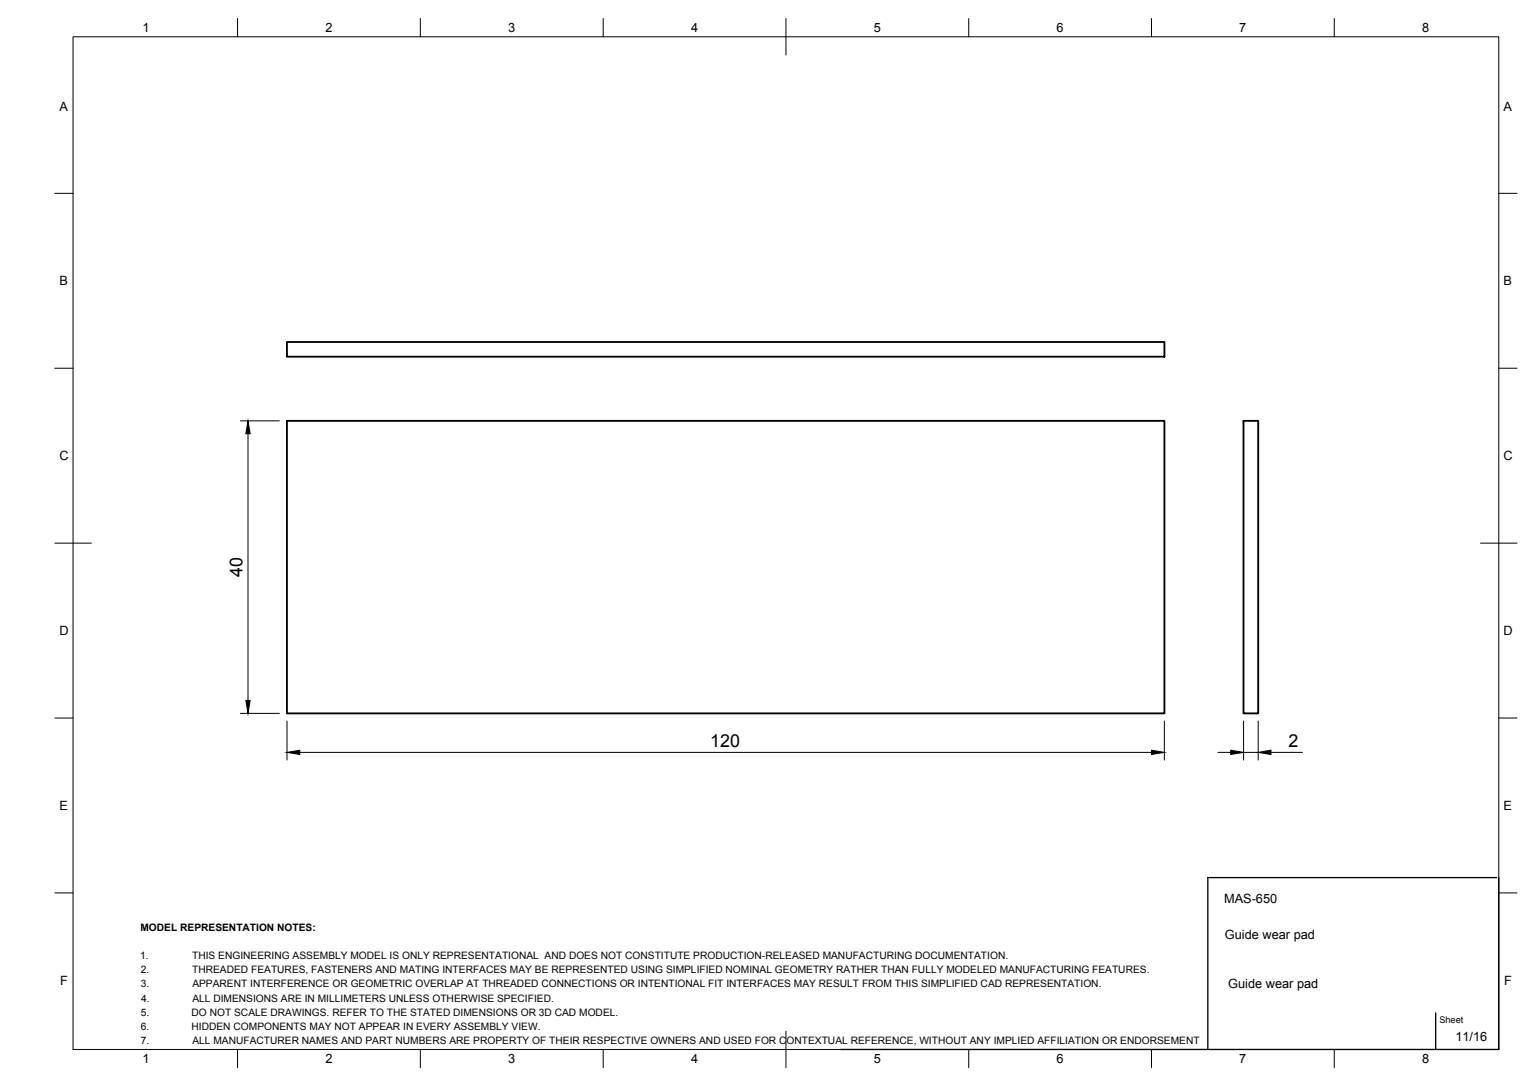
ISO-10303-21;
HEADER;
/* Generated by software containing ST-Developer
 * from STEP Tools, Inc. (www.steptools.com) 
 */

FILE_DESCRIPTION(
/* description */ ('Independent manual traversing gantry with native reusable aluminum pr
ofiles,180mm captured carriage travel, four bronze-bushed rollers, lin
ked ideal rolling motion, bonded acetal lateral guides, positive welde
d end stops and fully retained axle stacks. Editable native profile cu
t lengths220/400mm. Tool attachments viaM6 bridge-plate taps; mounted 
tool outside assembly. Welds, anchors, adhesives, fits, traction, load
/speed/structural/life ratings unassigned.'),
/* implementation_level */ '2;1');

FILE_NAME(
/* name */ 'Guide wear pad.step',
/* time_stamp */ '2026-11-09T20:04:38-08:00',
/* author */ (''),
/* organization */ (''),
/* preprocessor_version */ 'ST-DEVELOPER v20.2',
/* originating_system */ 'Autodesk Translation Framework v15.17.0.0',
/* authorisation */ '');

FILE_SCHEMA (('AUTOMOTIVE_DESIGN { 1 0 10303 214 3 1 1 }'));
ENDSEC;

DATA;
#10=MECHANICAL_DESIGN_GEOMETRIC_PRESENTATION_REPRESENTATION('',(#479),#13231);
#447=SHAPE_REPRESENTATION_RELATIONSHIP('SRR','None',#13336,#463);
#463=ADVANCED_BREP_SHAPE_REPRESENTATION('',(#495),#13223);
#479=STYLED_ITEM('',(#13424),#495);
#495=MANIFOLD_SOLID_BREP('Body1',#4159);
#608=PLANE('',#4598);
#609=PLANE('',#4599);
#610=PLANE('',#4600);
#611=PLANE('',#4601);
#612=PLANE('',#4602);
#613=PLANE('',#4603);
#813=FACE_OUTER_BOUND('',#1070,.T.);
#814=FACE_OUTER_BOUND('',#1071,.T.);
#815=FACE_OUTER_BOUND('',#1072,.T.);
#816=FACE_OUTER_BOUND('',#1073,.T.);
#817=FACE_OUTER_BOUND('',#1074,.T.);
#818=FACE_OUTER_BOUND('',#1075,.T.);
#1070=EDGE_LOOP('',(#3666,#3667,#3668,#3669));
#1071=EDGE_LOOP('',(#3670,#3671,#3672,#3673));
#1072=EDGE_LOOP('',(#3674,#3675,#3676,#3677));
#1073=EDGE_LOOP('',(#3678,#3679,#3680,#3681));
#1074=EDGE_LOOP('',(#3682,#3683,#3684,#3685));
#1075=EDGE_LOOP('',(#3686,#3687,#3688,#3689));
#1352=LINE('',#12984,#1614);
#1353=LINE('',#12986,#1615);
#1354=LINE('',#12988,#1616);
#1355=LINE('',#12989,#1617);
#1356=LINE('',#12992,#1618);
#1357=LINE('',#12994,#1619);
#1358=LINE('',#12995,#1620);
#1359=LINE('',#12998,#1621);
#1360=LINE('',#13000,#1622);
#1361=LINE('',#13001,#1623);
#1362=LINE('',#13003,#1624);
#1363=LINE('',#13004,#1625);
#1614=VECTOR('',#5473,10.);
#1615=VECTOR('',#5474,10.);
#1616=VECTOR('',#5475,10.);
#1617=VECTOR('',#5476,10.);
#1618=VECTOR('',#5479,10.);
#1619=VECTOR('',#5480,10.);
#1620=VECTOR('',#5481,10.);
#1621=VECTOR('',#5484,10.);
#1622=VECTOR('',#5485,10.);
#1623=VECTOR('',#5486,10.);
#1624=VECTOR('',#5489,10.);
#1625=VECTOR('',#5490,10.);
#2080=VERTEX_POINT('',#12982);
#2081=VERTEX_POINT('',#12983);
#2082=VERTEX_POINT('',#12985);
#2083=VERTEX_POINT('',#12987);
#2084=VERTEX_POINT('',#12991);
#2085=VERTEX_POINT('',#12993);
#2086=VERTEX_POINT('',#12997);
#2087=VERTEX_POINT('',#12999);
#2616=EDGE_CURVE('',#2080,#2081,#1352,.T.);
#2617=EDGE_CURVE('',#2081,#2082,#1353,.T.);
#2618=EDGE_CURVE('',#2083,#2082,#1354,.T.);
#2619=EDGE_CURVE('',#2080,#2083,#1355,.T.);
#2620=EDGE_CURVE('',#2084,#2080,#1356,.T.);
#2621=EDGE_CURVE('',#2085,#2083,#1357,.T.);
#2622=EDGE_CURVE('',#2084,#2085,#1358,.T.);
#2623=EDGE_CURVE('',#2086,#2084,#1359,.T.);
#2624=EDGE_CURVE('',#2087,#2085,#1360,.T.);
#2625=EDGE_CURVE('',#2086,#2087,#1361,.T.);
#2626=EDGE_CURVE('',#2081,#2086,#1362,.T.);
#2627=EDGE_CURVE('',#2082,#2087,#1363,.T.);
#3666=ORIENTED_EDGE('',*,*,#2616,.T.);
#3667=ORIENTED_EDGE('',*,*,#2617,.T.);
#3668=ORIENTED_EDGE('',*,*,#2618,.F.);
#3669=ORIENTED_EDGE('',*,*,#2619,.F.);
#3670=ORIENTED_EDGE('',*,*,#2620,.T.);
#3671=ORIENTED_EDGE('',*,*,#2619,.T.);
#3672=ORIENTED_EDGE('',*,*,#2621,.F.);
#3673=ORIENTED_EDGE('',*,*,#2622,.F.);
#3674=ORIENTED_EDGE('',*,*,#2623,.T.);
#3675=ORIENTED_EDGE('',*,*,#2622,.T.);
#3676=ORIENTED_EDGE('',*,*,#2624,.F.);
#3677=ORIENTED_EDGE('',*,*,#2625,.F.);
#3678=ORIENTED_EDGE('',*,*,#2626,.T.);
#3679=ORIENTED_EDGE('',*,*,#2625,.T.);
#3680=ORIENTED_EDGE('',*,*,#2627,.F.);
#3681=ORIENTED_EDGE('',*,*,#2617,.F.);
#3682=ORIENTED_EDGE('',*,*,#2627,.T.);
#3683=ORIENTED_EDGE('',*,*,#2624,.T.);
#3684=ORIENTED_EDGE('',*,*,#2621,.T.);
#3685=ORIENTED_EDGE('',*,*,#2618,.T.);
#3686=ORIENTED_EDGE('',*,*,#2626,.F.);
#3687=ORIENTED_EDGE('',*,*,#2616,.F.);
#3688=ORIENTED_EDGE('',*,*,#2620,.F.);
#3689=ORIENTED_EDGE('',*,*,#2623,.F.);
#4110=ADVANCED_FACE('',(#813),#608,.T.);
#4111=ADVANCED_FACE('',(#814),#609,.T.);
#4112=ADVANCED_FACE('',(#815),#610,.T.);
#4113=ADVANCED_FACE('',(#816),#611,.T.);
#4114=ADVANCED_FACE('',(#817),#612,.T.);
#4115=ADVANCED_FACE('',(#818),#613,.F.);
#4159=CLOSED_SHELL('',(#4110,#4111,#4112,#4113,#4114,#4115));
#4597=AXIS2_PLACEMENT_3D('',#12980,#5469,#5470);
#4598=AXIS2_PLACEMENT_3D('',#12981,#5471,#5472);
#4599=AXIS2_PLACEMENT_3D('',#12990,#5477,#5478);
#4600=AXIS2_PLACEMENT_3D('',#12996,#5482,#5483);
#4601=AXIS2_PLACEMENT_3D('',#13002,#5487,#5488);
#4602=AXIS2_PLACEMENT_3D('',#13005,#5491,#5492);
#4603=AXIS2_PLACEMENT_3D('',#13006,#5493,#5494);
#5469=DIRECTION('axis',(0.,0.,1.));
#5470=DIRECTION('refdir',(1.,0.,0.));
#5471=DIRECTION('center_axis',(0.,1.,0.));
#5472=DIRECTION('ref_axis',(-1.,0.,0.));
#5473=DIRECTION('',(-1.,0.,0.));
#5474=DIRECTION('',(0.,0.,1.));
#5475=DIRECTION('',(-1.,0.,0.));
#5476=DIRECTION('',(0.,0.,1.));
#5477=DIRECTION('center_axis',(1.,0.,0.));
#5478=DIRECTION('ref_axis',(0.,1.,0.));
#5479=DIRECTION('',(0.,1.,0.));
#5480=DIRECTION('',(0.,1.,0.));
#5481=DIRECTION('',(0.,0.,1.));
#5482=DIRECTION('center_axis',(0.,-1.,0.));
#5483=DIRECTION('ref_axis',(1.,0.,0.));
#5484=DIRECTION('',(1.,0.,0.));
#5485=DIRECTION('',(1.,0.,0.));
#5486=DIRECTION('',(0.,0.,1.));
#5487=DIRECTION('center_axis',(-1.,0.,0.));
#5488=DIRECTION('ref_axis',(0.,-1.,0.));
#5489=DIRECTION('',(0.,-1.,0.));
#5490=DIRECTION('',(0.,-1.,0.));
#5491=DIRECTION('center_axis',(0.,0.,1.));
#5492=DIRECTION('ref_axis',(1.,0.,0.));
#5493=DIRECTION('center_axis',(0.,0.,1.));
#5494=DIRECTION('ref_axis',(1.,0.,0.));
#12980=CARTESIAN_POINT('',(0.,0.,0.));
#12981=CARTESIAN_POINT('Origin',(60.,1.,240.));
#12982=CARTESIAN_POINT('',(60.,1.,240.));
#12983=CARTESIAN_POINT('',(-60.,1.,240.));
#12984=CARTESIAN_POINT('',(60.,1.,240.));
#12985=CARTESIAN_POINT('',(-60.,1.,280.));
#12986=CARTESIAN_POINT('',(-60.,1.,240.));
#12987=CARTESIAN_POINT('',(60.,1.,280.));
#12988=CARTESIAN_POINT('',(60.,1.,280.));
#12989=CARTESIAN_POINT('',(60.,1.,240.));
#12990=CARTESIAN_POINT('Origin',(60.,-1.,240.));
#12991=CARTESIAN_POINT('',(60.,-1.,240.));
#12992=CARTESIAN_POINT('',(60.,-1.,240.));
#12993=CARTESIAN_POINT('',(60.,-1.,280.));
#12994=CARTESIAN_POINT('',(60.,-1.,280.));
#12995=CARTESIAN_POINT('',(60.,-1.,240.));
#12996=CARTESIAN_POINT('Origin',(-60.,-1.,240.));
#12997=CARTESIAN_POINT('',(-60.,-1.,240.));
#12998=CARTESIAN_POINT('',(-60.,-1.,240.));
#12999=CARTESIAN_POINT('',(-60.,-1.,280.));
#13000=CARTESIAN_POINT('',(-60.,-1.,280.));
#13001=CARTESIAN_POINT('',(-60.,-1.,240.));
#13002=CARTESIAN_POINT('Origin',(-60.,1.,240.));
#13003=CARTESIAN_POINT('',(-60.,1.,240.));
#13004=CARTESIAN_POINT('',(-60.,1.,280.));
#13005=CARTESIAN_POINT('Origin',(0.,0.,280.));
#13006=CARTESIAN_POINT('Origin',(0.,0.,240.));
#13205=UNCERTAINTY_MEASURE_WITH_UNIT(LENGTH_MEASURE(0.01),#13232,
'DISTANCE_ACCURACY_VALUE',
'Maximum model space distance between geometric entities at asserted c
onnectivities');
#13213=UNCERTAINTY_MEASURE_WITH_UNIT(LENGTH_MEASURE(0.01),#13232,
'DISTANCE_ACCURACY_VALUE',
'Maximum model space distance between geometric entities at asserted c
onnectivities');
#13223=(
GEOMETRIC_REPRESENTATION_CONTEXT(3)
GLOBAL_UNCERTAINTY_ASSIGNED_CONTEXT((#13205))
GLOBAL_UNIT_ASSIGNED_CONTEXT((#13232,#13234,#13235))
REPRESENTATION_CONTEXT('','3D')
);
#13231=(
GEOMETRIC_REPRESENTATION_CONTEXT(3)
GLOBAL_UNCERTAINTY_ASSIGNED_CONTEXT((#13213))
GLOBAL_UNIT_ASSIGNED_CONTEXT((#13232,#13234,#13235))
REPRESENTATION_CONTEXT('','3D')
);
#13232=(
LENGTH_UNIT()
NAMED_UNIT(*)
SI_UNIT(.MILLI.,.METRE.)
);
#13234=(
NAMED_UNIT(*)
PLANE_ANGLE_UNIT()
SI_UNIT($,.RADIAN.)
);
#13235=(
NAMED_UNIT(*)
SI_UNIT($,.STERADIAN.)
SOLID_ANGLE_UNIT()
);
#13245=SHAPE_DEFINITION_REPRESENTATION(#13262,#13336);
#13262=PRODUCT_DEFINITION_SHAPE('',$,#13354);
#13336=SHAPE_REPRESENTATION('',(#4597),#13223);
#13344=PRODUCT_DEFINITION_CONTEXT('part definition',#13397,'design');
#13354=PRODUCT_DEFINITION('Guide wear pad','Guide wear pad',#13371,#13344);
#13371=PRODUCT_DEFINITION_FORMATION('',$,#13408);
#13397=APPLICATION_CONTEXT(
'Core Data for Automotive Mechanical Design Process');
#13398=PRODUCT_CONTEXT('part definition',#13397,'mechanical');
#13408=PRODUCT('Guide wear pad','Guide wear pad',$,(#13398));
#13424=PRESENTATION_STYLE_ASSIGNMENT((#13438));
#13438=SURFACE_STYLE_USAGE(.BOTH.,#13452);
#13452=SURFACE_SIDE_STYLE('',(#13466));
#13466=SURFACE_STYLE_FILL_AREA(#13480);
#13480=FILL_AREA_STYLE('Wear pad gray',(#13494));
#13494=FILL_AREA_STYLE_COLOUR('Wear pad gray',#13508);
#13508=COLOUR_RGB('Wear pad gray',0.725490196078431,0.752941176470588,0.792156862745098);
ENDSEC;
END-ISO-10303-21;
